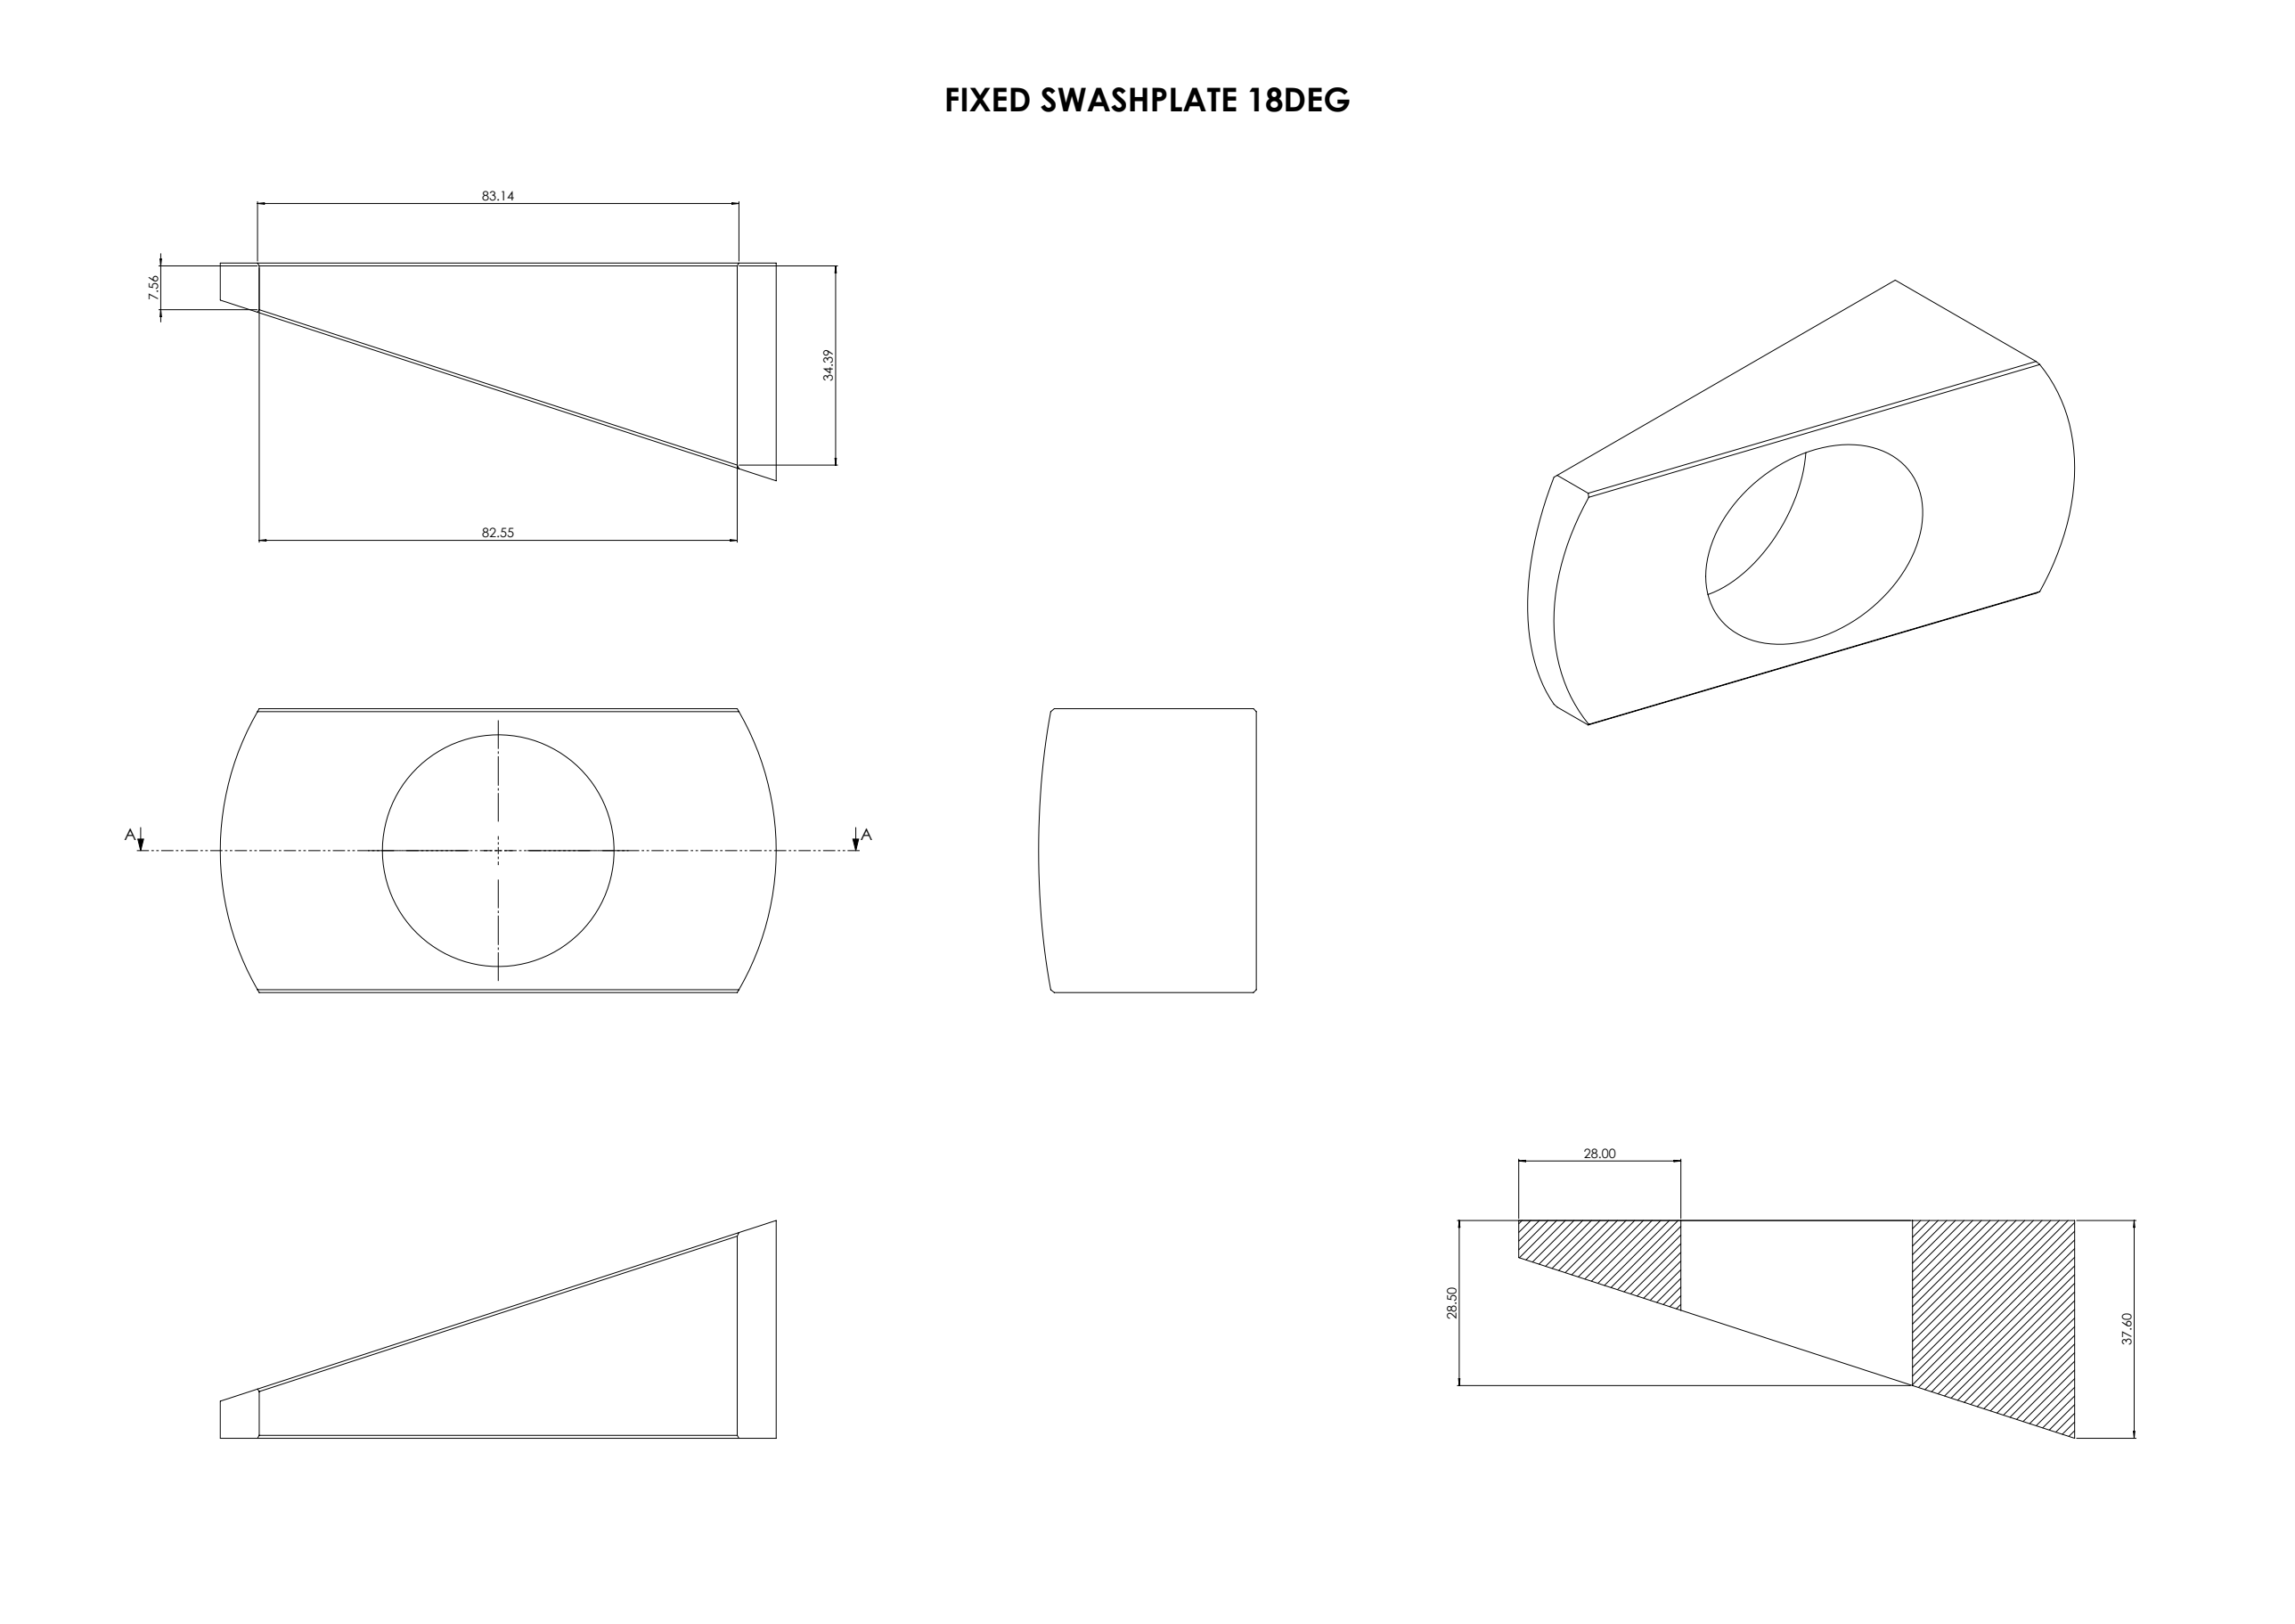
ISO-10303-21;
HEADER;
/* Generated by software containing ST-Developer
 * from STEP Tools, Inc. (www.steptools.com) 
 */

FILE_DESCRIPTION(
/* description */ (''),
/* implementation_level */ '2;1');

FILE_NAME(
/* name */ '03_Fixed_Swashplate_18deg.step',
/* time_stamp */ '2026-10-26T07:49:00-07:00',
/* author */ (''),
/* organization */ (''),
/* preprocessor_version */ 'ST-DEVELOPER v20.2',
/* originating_system */ 'Autodesk Translation Framework v15.15.0.0',
/* authorisation */ '');

FILE_SCHEMA (('AUTOMOTIVE_DESIGN { 1 0 10303 214 3 1 1 }'));
ENDSEC;

DATA;
#10=MECHANICAL_DESIGN_GEOMETRIC_PRESENTATION_REPRESENTATION('',(#179),#38507);
#149=SHAPE_REPRESENTATION_RELATIONSHIP('SRR','None',#38577,#164);
#164=ADVANCED_BREP_SHAPE_REPRESENTATION('',(#194),#38494);
#179=STYLED_ITEM('',(#38706),#194);
#194=MANIFOLD_SOLID_BREP('Body1',#15073);
#301=ELLIPSE('',#15801,67.8822509939087,48.);
#302=ELLIPSE('',#15802,67.8822509939087,48.);
#303=ELLIPSE('',#15806,67.8822509939087,48.);
#304=ELLIPSE('',#15807,71.3756226163554,48.);
#305=ELLIPSE('',#15808,50.4701867634368,48.);
#306=ELLIPSE('',#15809,71.3756226163554,48.);
#307=ELLIPSE('',#15811,71.3756226163554,48.);
#308=ELLIPSE('',#15813,50.4701867634368,48.);
#309=ELLIPSE('',#15814,21.0292444847653,20.);
#310=ELLIPSE('',#15816,67.8822509939087,48.);
#311=ELLIPSE('',#15821,71.3756226163554,48.);
#455=FACE_BOUND('',#2841,.T.);
#456=FACE_BOUND('',#2844,.T.);
#626=PLANE('',#15800);
#627=PLANE('',#15803);
#628=PLANE('',#15810);
#629=PLANE('',#15812);
#630=PLANE('',#15815);
#631=PLANE('',#15817);
#632=PLANE('',#15820);
#633=PLANE('',#15824);
#1464=CYLINDRICAL_SURFACE('',#15804,48.);
#1465=CYLINDRICAL_SURFACE('',#15822,48.);
#1466=CYLINDRICAL_SURFACE('',#15823,20.);
#1911=FACE_OUTER_BOUND('',#2836,.T.);
#1912=FACE_OUTER_BOUND('',#2837,.T.);
#1913=FACE_OUTER_BOUND('',#2838,.T.);
#1914=FACE_OUTER_BOUND('',#2839,.T.);
#1915=FACE_OUTER_BOUND('',#2840,.T.);
#1916=FACE_OUTER_BOUND('',#2842,.T.);
#1917=FACE_OUTER_BOUND('',#2843,.T.);
#1918=FACE_OUTER_BOUND('',#2845,.T.);
#1919=FACE_OUTER_BOUND('',#2846,.T.);
#1920=FACE_OUTER_BOUND('',#2847,.T.);
#1921=FACE_OUTER_BOUND('',#2848,.T.);
#2836=EDGE_LOOP('',(#11183,#11184,#11185,#11186));
#2837=EDGE_LOOP('',(#11187,#11188,#11189,#11190));
#2838=EDGE_LOOP('',(#11191,#11192,#11193,#11194,#11195,#11196,#11197,#11198));
#2839=EDGE_LOOP('',(#11199,#11200,#11201,#11202));
#2840=EDGE_LOOP('',(#11203,#11204,#11205,#11206));
#2841=EDGE_LOOP('',(#11207));
#2842=EDGE_LOOP('',(#11208,#11209,#11210,#11211));
#2843=EDGE_LOOP('',(#11212,#11213,#11214,#11215));
#2844=EDGE_LOOP('',(#11216));
#2845=EDGE_LOOP('',(#11217,#11218,#11219,#11220));
#2846=EDGE_LOOP('',(#11221,#11222,#11223,#11224,#11225,#11226,#11227,#11228));
#2847=EDGE_LOOP('',(#11229,#11230,#11231,#11232));
#2848=EDGE_LOOP('',(#11233,#11234,#11235,#11236));
#3770=LINE('',#25417,#4839);
#3771=LINE('',#25420,#4840);
#3772=LINE('',#25423,#4841);
#3773=LINE('',#25425,#4842);
#3774=LINE('',#25426,#4843);
#3775=LINE('',#25433,#4844);
#3776=LINE('',#25442,#4845);
#3777=LINE('',#25445,#4846);
#3778=LINE('',#25453,#4847);
#3779=LINE('',#25454,#4848);
#3780=LINE('',#25461,#4849);
#3781=LINE('',#25464,#4850);
#3782=LINE('',#25466,#4851);
#4839=VECTOR('',#18113,10.);
#4840=VECTOR('',#18116,10.);
#4841=VECTOR('',#18119,10.);
#4842=VECTOR('',#18120,10.);
#4843=VECTOR('',#18121,10.);
#4844=VECTOR('',#18128,10.);
#4845=VECTOR('',#18139,10.);
#4846=VECTOR('',#18142,10.);
#4847=VECTOR('',#18151,10.);
#4848=VECTOR('',#18152,10.);
#4849=VECTOR('',#18161,10.);
#4850=VECTOR('',#18166,10.);
#4851=VECTOR('',#18169,20.);
#5957=CIRCLE('',#15805,48.);
#5958=CIRCLE('',#15818,48.);
#5959=CIRCLE('',#15819,20.);
#6689=VERTEX_POINT('',#25413);
#6690=VERTEX_POINT('',#25414);
#6691=VERTEX_POINT('',#25416);
#6692=VERTEX_POINT('',#25418);
#6693=VERTEX_POINT('',#25422);
#6694=VERTEX_POINT('',#25424);
#6695=VERTEX_POINT('',#25428);
#6696=VERTEX_POINT('',#25430);
#6697=VERTEX_POINT('',#25432);
#6698=VERTEX_POINT('',#25434);
#6699=VERTEX_POINT('',#25436);
#6700=VERTEX_POINT('',#25440);
#6701=VERTEX_POINT('',#25444);
#6702=VERTEX_POINT('',#25447);
#6703=VERTEX_POINT('',#25450);
#6704=VERTEX_POINT('',#25451);
#6705=VERTEX_POINT('',#25457);
#6706=VERTEX_POINT('',#25460);
#8340=EDGE_CURVE('',#6689,#6690,#301,.T.);
#8341=EDGE_CURVE('',#6690,#6691,#3770,.T.);
#8342=EDGE_CURVE('',#6691,#6692,#302,.T.);
#8343=EDGE_CURVE('',#6692,#6689,#3771,.T.);
#8344=EDGE_CURVE('',#6690,#6693,#3772,.T.);
#8345=EDGE_CURVE('',#6694,#6693,#3773,.T.);
#8346=EDGE_CURVE('',#6694,#6691,#3774,.T.);
#8347=EDGE_CURVE('',#6695,#6689,#5957,.T.);
#8348=EDGE_CURVE('',#6696,#6695,#303,.T.);
#8349=EDGE_CURVE('',#6697,#6696,#3775,.T.);
#8350=EDGE_CURVE('',#6698,#6697,#304,.T.);
#8351=EDGE_CURVE('',#6699,#6698,#305,.T.);
#8352=EDGE_CURVE('',#6693,#6699,#306,.T.);
#8353=EDGE_CURVE('',#6700,#6694,#307,.T.);
#8354=EDGE_CURVE('',#6699,#6700,#3776,.T.);
#8355=EDGE_CURVE('',#6701,#6698,#3777,.T.);
#8356=EDGE_CURVE('',#6701,#6700,#308,.T.);
#8357=EDGE_CURVE('',#6702,#6702,#309,.T.);
#8358=EDGE_CURVE('',#6703,#6704,#310,.T.);
#8359=EDGE_CURVE('',#6704,#6696,#3778,.T.);
#8360=EDGE_CURVE('',#6695,#6703,#3779,.T.);
#8361=EDGE_CURVE('',#6692,#6703,#5958,.T.);
#8362=EDGE_CURVE('',#6705,#6705,#5959,.T.);
#8363=EDGE_CURVE('',#6697,#6706,#3780,.T.);
#8364=EDGE_CURVE('',#6706,#6701,#311,.T.);
#8365=EDGE_CURVE('',#6704,#6706,#3781,.T.);
#8366=EDGE_CURVE('',#6705,#6702,#3782,.T.);
#11183=ORIENTED_EDGE('',*,*,#8340,.T.);
#11184=ORIENTED_EDGE('',*,*,#8341,.T.);
#11185=ORIENTED_EDGE('',*,*,#8342,.T.);
#11186=ORIENTED_EDGE('',*,*,#8343,.T.);
#11187=ORIENTED_EDGE('',*,*,#8341,.F.);
#11188=ORIENTED_EDGE('',*,*,#8344,.T.);
#11189=ORIENTED_EDGE('',*,*,#8345,.F.);
#11190=ORIENTED_EDGE('',*,*,#8346,.T.);
#11191=ORIENTED_EDGE('',*,*,#8340,.F.);
#11192=ORIENTED_EDGE('',*,*,#8347,.F.);
#11193=ORIENTED_EDGE('',*,*,#8348,.F.);
#11194=ORIENTED_EDGE('',*,*,#8349,.F.);
#11195=ORIENTED_EDGE('',*,*,#8350,.F.);
#11196=ORIENTED_EDGE('',*,*,#8351,.F.);
#11197=ORIENTED_EDGE('',*,*,#8352,.F.);
#11198=ORIENTED_EDGE('',*,*,#8344,.F.);
#11199=ORIENTED_EDGE('',*,*,#8353,.T.);
#11200=ORIENTED_EDGE('',*,*,#8345,.T.);
#11201=ORIENTED_EDGE('',*,*,#8352,.T.);
#11202=ORIENTED_EDGE('',*,*,#8354,.T.);
#11203=ORIENTED_EDGE('',*,*,#8354,.F.);
#11204=ORIENTED_EDGE('',*,*,#8351,.T.);
#11205=ORIENTED_EDGE('',*,*,#8355,.F.);
#11206=ORIENTED_EDGE('',*,*,#8356,.T.);
#11207=ORIENTED_EDGE('',*,*,#8357,.T.);
#11208=ORIENTED_EDGE('',*,*,#8358,.T.);
#11209=ORIENTED_EDGE('',*,*,#8359,.T.);
#11210=ORIENTED_EDGE('',*,*,#8348,.T.);
#11211=ORIENTED_EDGE('',*,*,#8360,.T.);
#11212=ORIENTED_EDGE('',*,*,#8343,.F.);
#11213=ORIENTED_EDGE('',*,*,#8361,.T.);
#11214=ORIENTED_EDGE('',*,*,#8360,.F.);
#11215=ORIENTED_EDGE('',*,*,#8347,.T.);
#11216=ORIENTED_EDGE('',*,*,#8362,.T.);
#11217=ORIENTED_EDGE('',*,*,#8350,.T.);
#11218=ORIENTED_EDGE('',*,*,#8363,.T.);
#11219=ORIENTED_EDGE('',*,*,#8364,.T.);
#11220=ORIENTED_EDGE('',*,*,#8355,.T.);
#11221=ORIENTED_EDGE('',*,*,#8342,.F.);
#11222=ORIENTED_EDGE('',*,*,#8346,.F.);
#11223=ORIENTED_EDGE('',*,*,#8353,.F.);
#11224=ORIENTED_EDGE('',*,*,#8356,.F.);
#11225=ORIENTED_EDGE('',*,*,#8364,.F.);
#11226=ORIENTED_EDGE('',*,*,#8365,.F.);
#11227=ORIENTED_EDGE('',*,*,#8358,.F.);
#11228=ORIENTED_EDGE('',*,*,#8361,.F.);
#11229=ORIENTED_EDGE('',*,*,#8362,.F.);
#11230=ORIENTED_EDGE('',*,*,#8366,.T.);
#11231=ORIENTED_EDGE('',*,*,#8357,.F.);
#11232=ORIENTED_EDGE('',*,*,#8366,.F.);
#11233=ORIENTED_EDGE('',*,*,#8359,.F.);
#11234=ORIENTED_EDGE('',*,*,#8365,.T.);
#11235=ORIENTED_EDGE('',*,*,#8363,.F.);
#11236=ORIENTED_EDGE('',*,*,#8349,.T.);
#14478=ADVANCED_FACE('',(#1911),#626,.T.);
#14479=ADVANCED_FACE('',(#1912),#627,.T.);
#14480=ADVANCED_FACE('',(#1913),#1464,.T.);
#14481=ADVANCED_FACE('',(#1914),#628,.T.);
#14482=ADVANCED_FACE('',(#1915,#455),#629,.T.);
#14483=ADVANCED_FACE('',(#1916),#630,.T.);
#14484=ADVANCED_FACE('',(#1917,#456),#631,.T.);
#14485=ADVANCED_FACE('',(#1918),#632,.T.);
#14486=ADVANCED_FACE('',(#1919),#1465,.T.);
#14487=ADVANCED_FACE('',(#1920),#1466,.F.);
#14488=ADVANCED_FACE('',(#1921),#633,.T.);
#15073=CLOSED_SHELL('',(#14478,#14479,#14480,#14481,#14482,#14483,#14484,
#14485,#14486,#14487,#14488));
#15799=AXIS2_PLACEMENT_3D('',#25411,#18107,#18108);
#15800=AXIS2_PLACEMENT_3D('',#25412,#18109,#18110);
#15801=AXIS2_PLACEMENT_3D('',#25415,#18111,#18112);
#15802=AXIS2_PLACEMENT_3D('',#25419,#18114,#18115);
#15803=AXIS2_PLACEMENT_3D('',#25421,#18117,#18118);
#15804=AXIS2_PLACEMENT_3D('',#25427,#18122,#18123);
#15805=AXIS2_PLACEMENT_3D('',#25429,#18124,#18125);
#15806=AXIS2_PLACEMENT_3D('',#25431,#18126,#18127);
#15807=AXIS2_PLACEMENT_3D('',#25435,#18129,#18130);
#15808=AXIS2_PLACEMENT_3D('',#25437,#18131,#18132);
#15809=AXIS2_PLACEMENT_3D('',#25438,#18133,#18134);
#15810=AXIS2_PLACEMENT_3D('',#25439,#18135,#18136);
#15811=AXIS2_PLACEMENT_3D('',#25441,#18137,#18138);
#15812=AXIS2_PLACEMENT_3D('',#25443,#18140,#18141);
#15813=AXIS2_PLACEMENT_3D('',#25446,#18143,#18144);
#15814=AXIS2_PLACEMENT_3D('',#25448,#18145,#18146);
#15815=AXIS2_PLACEMENT_3D('',#25449,#18147,#18148);
#15816=AXIS2_PLACEMENT_3D('',#25452,#18149,#18150);
#15817=AXIS2_PLACEMENT_3D('',#25455,#18153,#18154);
#15818=AXIS2_PLACEMENT_3D('',#25456,#18155,#18156);
#15819=AXIS2_PLACEMENT_3D('',#25458,#18157,#18158);
#15820=AXIS2_PLACEMENT_3D('',#25459,#18159,#18160);
#15821=AXIS2_PLACEMENT_3D('',#25462,#18162,#18163);
#15822=AXIS2_PLACEMENT_3D('',#25463,#18164,#18165);
#15823=AXIS2_PLACEMENT_3D('',#25465,#18167,#18168);
#15824=AXIS2_PLACEMENT_3D('',#25467,#18170,#18171);
#18107=DIRECTION('axis',(0.,0.,1.));
#18108=DIRECTION('refdir',(1.,0.,0.));
#18109=DIRECTION('center_axis',(-0.707106781186546,-0.707106781186549,0.));
#18110=DIRECTION('ref_axis',(0.,0.,1.));
#18111=DIRECTION('center_axis',(-0.707106781186546,-0.707106781186549,0.));
#18112=DIRECTION('ref_axis',(-0.707106781186549,0.707106781186546,0.));
#18113=DIRECTION('',(0.,0.,1.));
#18114=DIRECTION('center_axis',(-0.707106781186546,-0.707106781186549,0.));
#18115=DIRECTION('ref_axis',(-0.707106781186549,0.707106781186546,0.));
#18116=DIRECTION('',(0.,0.,-1.));
#18117=DIRECTION('center_axis',(0.,-1.,0.));
#18118=DIRECTION('ref_axis',(0.,0.,-1.));
#18119=DIRECTION('',(1.,0.,0.));
#18120=DIRECTION('',(0.309016994374947,0.,-0.951056516295154));
#18121=DIRECTION('',(-1.,0.,0.));
#18122=DIRECTION('center_axis',(1.,0.,0.));
#18123=DIRECTION('ref_axis',(0.,1.,0.));
#18124=DIRECTION('center_axis',(-1.,0.,0.));
#18125=DIRECTION('ref_axis',(0.,1.,0.));
#18126=DIRECTION('center_axis',(-0.707106781186546,0.707106781186549,0.));
#18127=DIRECTION('ref_axis',(0.707106781186549,0.707106781186546,0.));
#18128=DIRECTION('',(-1.,0.,0.));
#18129=DIRECTION('center_axis',(0.672498511963957,0.707106781186548,0.21850801222441));
#18130=DIRECTION('ref_axis',(-0.740098474127776,0.6425202520624,0.198549677117357));
#18131=DIRECTION('center_axis',(0.951056516295154,0.,0.309016994374947));
#18132=DIRECTION('ref_axis',(-0.309016994374947,0.,0.951056516295154));
#18133=DIRECTION('center_axis',(0.672498511963957,-0.707106781186548,0.21850801222441));
#18134=DIRECTION('ref_axis',(0.740098474127776,0.6425202520624,-0.198549677117357));
#18135=DIRECTION('center_axis',(0.672498511963957,-0.707106781186548,0.21850801222441));
#18136=DIRECTION('ref_axis',(0.309016994374947,0.,-0.951056516295154));
#18137=DIRECTION('center_axis',(0.672498511963957,-0.707106781186548,0.21850801222441));
#18138=DIRECTION('ref_axis',(0.740098474127776,0.6425202520624,-0.198549677117357));
#18139=DIRECTION('',(-0.309016994374947,0.,0.951056516295154));
#18140=DIRECTION('center_axis',(0.951056516295154,0.,0.309016994374947));
#18141=DIRECTION('ref_axis',(0.309016994374947,0.,-0.951056516295154));
#18142=DIRECTION('',(0.309016994374947,0.,-0.951056516295154));
#18143=DIRECTION('center_axis',(0.951056516295154,0.,0.309016994374947));
#18144=DIRECTION('ref_axis',(-0.309016994374947,0.,0.951056516295154));
#18145=DIRECTION('center_axis',(-0.951056516295154,0.,-0.309016994374947));
#18146=DIRECTION('ref_axis',(-0.309016994374947,0.,0.951056516295154));
#18147=DIRECTION('center_axis',(-0.707106781186546,0.707106781186549,0.));
#18148=DIRECTION('ref_axis',(0.,0.,1.));
#18149=DIRECTION('center_axis',(-0.707106781186546,0.707106781186549,0.));
#18150=DIRECTION('ref_axis',(0.707106781186549,0.707106781186546,0.));
#18151=DIRECTION('',(0.,0.,-1.));
#18152=DIRECTION('',(0.,0.,1.));
#18153=DIRECTION('center_axis',(-1.,0.,0.));
#18154=DIRECTION('ref_axis',(0.,0.,1.));
#18155=DIRECTION('center_axis',(-1.,0.,0.));
#18156=DIRECTION('ref_axis',(0.,1.,0.));
#18157=DIRECTION('center_axis',(1.,0.,0.));
#18158=DIRECTION('ref_axis',(0.,1.,0.));
#18159=DIRECTION('center_axis',(0.672498511963957,0.707106781186548,0.21850801222441));
#18160=DIRECTION('ref_axis',(0.309016994374947,0.,-0.951056516295154));
#18161=DIRECTION('',(-0.309016994374947,0.,0.951056516295154));
#18162=DIRECTION('center_axis',(0.672498511963957,0.707106781186548,0.21850801222441));
#18163=DIRECTION('ref_axis',(-0.740098474127776,0.6425202520624,0.198549677117357));
#18164=DIRECTION('center_axis',(1.,0.,0.));
#18165=DIRECTION('ref_axis',(0.,1.,0.));
#18166=DIRECTION('',(1.,0.,0.));
#18167=DIRECTION('center_axis',(1.,0.,0.));
#18168=DIRECTION('ref_axis',(0.,1.,0.));
#18169=DIRECTION('',(1.,0.,0.));
#18170=DIRECTION('center_axis',(0.,1.,0.));
#18171=DIRECTION('ref_axis',(0.,0.,1.));
#25411=CARTESIAN_POINT('',(0.,0.,0.));
#25412=CARTESIAN_POINT('Origin',(16.25,-24.25,-24.5));
#25413=CARTESIAN_POINT('',(16.,-24.,-41.569219381653));
#25414=CARTESIAN_POINT('',(16.5,-24.5,-41.2765066351308));
#25415=CARTESIAN_POINT('Origin',(-8.0000000000001,0.,0.));
#25416=CARTESIAN_POINT('',(16.5,-24.5,41.2765066351308));
#25417=CARTESIAN_POINT('',(16.5,-24.5,-24.5));
#25418=CARTESIAN_POINT('',(16.,-24.,41.569219381653));
#25419=CARTESIAN_POINT('Origin',(-8.0000000000001,0.,0.));
#25420=CARTESIAN_POINT('',(16.,-24.,-24.5));
#25421=CARTESIAN_POINT('Origin',(34.9605325577062,-24.5,0.));
#25422=CARTESIAN_POINT('',(50.8858188853231,-24.5,-41.2765066351308));
#25423=CARTESIAN_POINT('',(42.5,-24.5,-41.2765066351308));
#25424=CARTESIAN_POINT('',(24.0627188904386,-24.5,41.2765066351308));
#25425=CARTESIAN_POINT('',(29.418817527239,-24.5,24.7921300371634));
#25426=CARTESIAN_POINT('',(42.5,-24.5,41.2765066351308));
#25427=CARTESIAN_POINT('Origin',(42.5,0.,0.));
#25428=CARTESIAN_POINT('',(16.,24.,-41.569219381653));
#25429=CARTESIAN_POINT('Origin',(16.,0.,0.));
#25430=CARTESIAN_POINT('',(16.5,24.5,-41.2765066351308));
#25431=CARTESIAN_POINT('Origin',(-8.0000000000001,0.,0.));
#25432=CARTESIAN_POINT('',(50.8858188853231,24.5,-41.2765066351308));
#25433=CARTESIAN_POINT('',(42.5,24.5,-41.2765066351308));
#25434=CARTESIAN_POINT('',(51.5066581341257,24.,-41.569219381653));
#25435=CARTESIAN_POINT('Origin',(63.2350933817184,0.,0.));
#25436=CARTESIAN_POINT('',(51.5066581341257,-24.,-41.569219381653));
#25437=CARTESIAN_POINT('Origin',(38.,0.,0.));
#25438=CARTESIAN_POINT('Origin',(63.2350933817184,0.,0.));
#25439=CARTESIAN_POINT('Origin',(29.6565816563128,-24.25,24.8693842857571));
#25440=CARTESIAN_POINT('',(24.4933418658742,-24.,41.569219381653));
#25441=CARTESIAN_POINT('Origin',(63.2350933817184,0.,0.));
#25442=CARTESIAN_POINT('',(29.8943457853866,-24.,24.9466385343509));
#25443=CARTESIAN_POINT('Origin',(22.0789348845876,0.,49.));
#25444=CARTESIAN_POINT('',(24.4933418658742,24.,41.569219381653));
#25445=CARTESIAN_POINT('',(29.8943457853866,24.,24.9466385343509));
#25446=CARTESIAN_POINT('Origin',(38.,0.,0.));
#25447=CARTESIAN_POINT('',(38.,-20.,-4.83914384121483E-15));
#25448=CARTESIAN_POINT('Origin',(38.,0.,0.));
#25449=CARTESIAN_POINT('Origin',(16.25,24.25,-24.5));
#25450=CARTESIAN_POINT('',(16.,24.,41.569219381653));
#25451=CARTESIAN_POINT('',(16.5,24.5,41.2765066351308));
#25452=CARTESIAN_POINT('Origin',(-8.0000000000001,0.,0.));
#25453=CARTESIAN_POINT('',(16.5,24.5,-24.5));
#25454=CARTESIAN_POINT('',(16.,24.,-24.5));
#25455=CARTESIAN_POINT('Origin',(16.,0.,-49.));
#25456=CARTESIAN_POINT('Origin',(16.,0.,0.));
#25457=CARTESIAN_POINT('',(16.,-20.,-2.44929359829471E-15));
#25458=CARTESIAN_POINT('Origin',(16.,0.,0.));
#25459=CARTESIAN_POINT('Origin',(29.6565816563128,24.25,24.8693842857571));
#25460=CARTESIAN_POINT('',(24.0627188904386,24.5,41.2765066351308));
#25461=CARTESIAN_POINT('',(29.418817527239,24.5,24.7921300371634));
#25462=CARTESIAN_POINT('Origin',(63.2350933817184,0.,0.));
#25463=CARTESIAN_POINT('Origin',(42.5,0.,0.));
#25464=CARTESIAN_POINT('',(42.5,24.5,41.2765066351308));
#25465=CARTESIAN_POINT('Origin',(42.5,0.,0.));
#25466=CARTESIAN_POINT('',(42.5,-20.,-2.44929359829471E-15));
#25467=CARTESIAN_POINT('Origin',(34.9605325577062,24.5,0.));
#38477=UNCERTAINTY_MEASURE_WITH_UNIT(LENGTH_MEASURE(0.01),#38508,
'DISTANCE_ACCURACY_VALUE',
'Maximum model space distance between geometric entities at asserted c
onnectivities');
#38490=UNCERTAINTY_MEASURE_WITH_UNIT(LENGTH_MEASURE(0.01),#38508,
'DISTANCE_ACCURACY_VALUE',
'Maximum model space distance between geometric entities at asserted c
onnectivities');
#38494=(
GEOMETRIC_REPRESENTATION_CONTEXT(3)
GLOBAL_UNCERTAINTY_ASSIGNED_CONTEXT((#38477))
GLOBAL_UNIT_ASSIGNED_CONTEXT((#38508,#38510,#38511))
REPRESENTATION_CONTEXT('','3D')
);
#38507=(
GEOMETRIC_REPRESENTATION_CONTEXT(3)
GLOBAL_UNCERTAINTY_ASSIGNED_CONTEXT((#38490))
GLOBAL_UNIT_ASSIGNED_CONTEXT((#38508,#38510,#38511))
REPRESENTATION_CONTEXT('','3D')
);
#38508=(
LENGTH_UNIT()
NAMED_UNIT(*)
SI_UNIT(.MILLI.,.METRE.)
);
#38510=(
NAMED_UNIT(*)
PLANE_ANGLE_UNIT()
SI_UNIT($,.RADIAN.)
);
#38511=(
NAMED_UNIT(*)
SI_UNIT($,.STERADIAN.)
SOLID_ANGLE_UNIT()
);
#38515=SHAPE_DEFINITION_REPRESENTATION(#38531,#38577);
#38531=PRODUCT_DEFINITION_SHAPE('',$,#38594);
#38577=SHAPE_REPRESENTATION('',(#15799),#38494);
#38590=PRODUCT_DEFINITION_CONTEXT('part definition',#38640,'design');
#38594=PRODUCT_DEFINITION('2026-10-26-01-10-46-042',
'03_Fixed_Swashplate_18deg',#38610,#38590);
#38610=PRODUCT_DEFINITION_FORMATION('',$,#38645);
#38640=APPLICATION_CONTEXT(
'Core Data for Automotive Mechanical Design Process');
#38641=PRODUCT_CONTEXT('part definition',#38640,'mechanical');
#38645=PRODUCT('2026-10-26-01-10-46-042','03_Fixed_Swashplate_18deg',$,
(#38641));
#38700=COLOUR_RGB('Light Blue',0.38,0.62,0.78);
#38701=FILL_AREA_STYLE_COLOUR('',#38700);
#38702=FILL_AREA_STYLE('',(#38701));
#38703=SURFACE_STYLE_FILL_AREA(#38702);
#38704=SURFACE_SIDE_STYLE('',(#38703));
#38705=SURFACE_STYLE_USAGE(.BOTH.,#38704);
#38706=PRESENTATION_STYLE_ASSIGNMENT((#38705));
ENDSEC;
END-ISO-10303-21;
